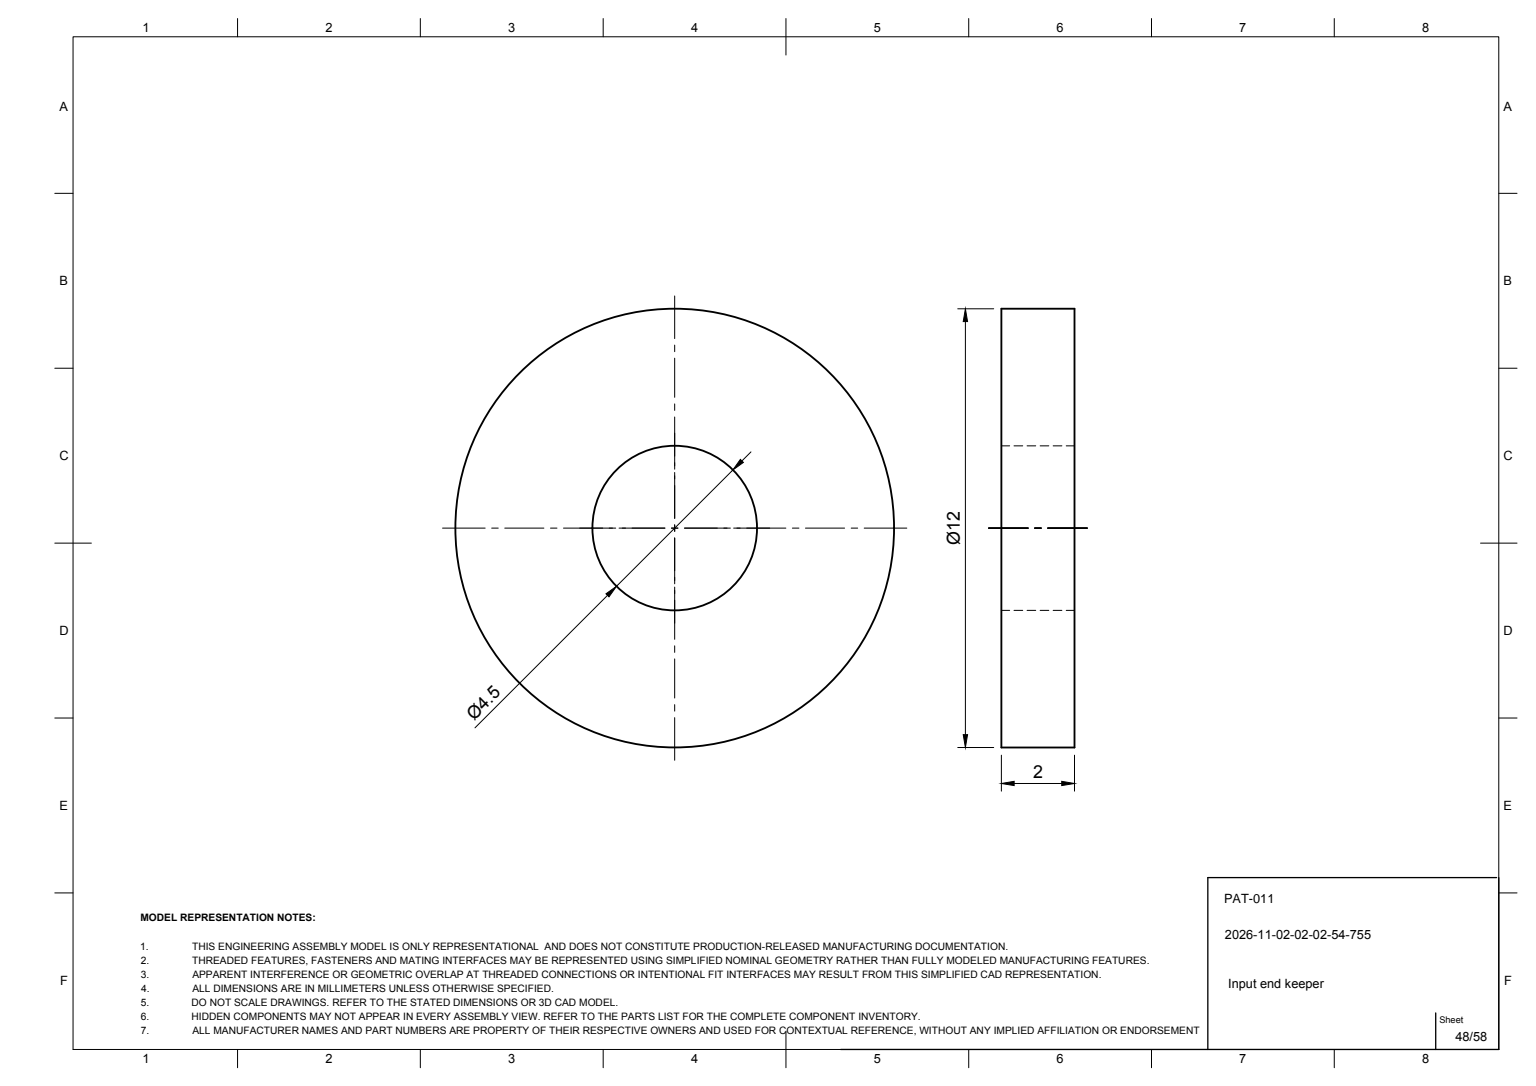
ISO-10303-21;
HEADER;
/* Generated by software containing ST-Developer
 * from STEP Tools, Inc. (www.steptools.com) 
 */

FILE_DESCRIPTION(
/* description */ ('Belt tension measurement rig'),
/* implementation_level */ '2;1');

FILE_NAME(
/* name */ 'Input end keeper.step',
/* time_stamp */ '2026-10-28T03:24:44-07:00',
/* author */ (''),
/* organization */ (''),
/* preprocessor_version */ 'ST-DEVELOPER v20.2',
/* originating_system */ 'Autodesk Translation Framework v15.17.0.0',
/* authorisation */ '');

FILE_SCHEMA (('AUTOMOTIVE_DESIGN { 1 0 10303 214 3 1 1 }'));
ENDSEC;

DATA;
#10=MECHANICAL_DESIGN_GEOMETRIC_PRESENTATION_REPRESENTATION('',(#749),#23587);
#624=SHAPE_REPRESENTATION_RELATIONSHIP('SRR','None',#23874,#679);
#679=ADVANCED_BREP_SHAPE_REPRESENTATION('',(#817),#23572);
#749=STYLED_ITEM('',(#24204),#817);
#817=MANIFOLD_SOLID_BREP('Body1',#12256);
#993=FACE_BOUND('',#2697,.T.);
#994=FACE_BOUND('',#2699,.T.);
#1292=PLANE('',#13869);
#1293=PLANE('',#13870);
#1826=FACE_OUTER_BOUND('',#2694,.T.);
#1827=FACE_OUTER_BOUND('',#2695,.T.);
#1828=FACE_OUTER_BOUND('',#2696,.T.);
#1829=FACE_OUTER_BOUND('',#2698,.T.);
#2694=EDGE_LOOP('',(#9992,#9993,#9994,#9995));
#2695=EDGE_LOOP('',(#9996,#9997,#9998,#9999));
#2696=EDGE_LOOP('',(#10000));
#2697=EDGE_LOOP('',(#10001));
#2698=EDGE_LOOP('',(#10002));
#2699=EDGE_LOOP('',(#10003));
#3505=LINE('',#21539,#4256);
#3506=LINE('',#21545,#4257);
#4256=VECTOR('',#17032,0.225);
#4257=VECTOR('',#17039,0.6);
#4920=CIRCLE('',#13864,0.225);
#4921=CIRCLE('',#13865,0.225);
#4922=CIRCLE('',#13867,0.6);
#4923=CIRCLE('',#13868,0.6);
#5935=VERTEX_POINT('',#21536);
#5936=VERTEX_POINT('',#21538);
#5937=VERTEX_POINT('',#21542);
#5938=VERTEX_POINT('',#21544);
#7355=EDGE_CURVE('',#5935,#5935,#4920,.T.);
#7356=EDGE_CURVE('',#5935,#5936,#3505,.T.);
#7357=EDGE_CURVE('',#5936,#5936,#4921,.T.);
#7358=EDGE_CURVE('',#5937,#5937,#4922,.T.);
#7359=EDGE_CURVE('',#5937,#5938,#3506,.T.);
#7360=EDGE_CURVE('',#5938,#5938,#4923,.T.);
#9992=ORIENTED_EDGE('',*,*,#7355,.F.);
#9993=ORIENTED_EDGE('',*,*,#7356,.T.);
#9994=ORIENTED_EDGE('',*,*,#7357,.T.);
#9995=ORIENTED_EDGE('',*,*,#7356,.F.);
#9996=ORIENTED_EDGE('',*,*,#7358,.F.);
#9997=ORIENTED_EDGE('',*,*,#7359,.T.);
#9998=ORIENTED_EDGE('',*,*,#7360,.T.);
#9999=ORIENTED_EDGE('',*,*,#7359,.F.);
#10000=ORIENTED_EDGE('',*,*,#7358,.T.);
#10001=ORIENTED_EDGE('',*,*,#7355,.T.);
#10002=ORIENTED_EDGE('',*,*,#7360,.F.);
#10003=ORIENTED_EDGE('',*,*,#7357,.F.);
#11329=CYLINDRICAL_SURFACE('',#13863,0.225);
#11330=CYLINDRICAL_SURFACE('',#13866,0.6);
#11967=ADVANCED_FACE('',(#1826),#11329,.F.);
#11968=ADVANCED_FACE('',(#1827),#11330,.T.);
#11969=ADVANCED_FACE('',(#1828,#993),#1292,.T.);
#11970=ADVANCED_FACE('',(#1829,#994),#1293,.F.);
#12256=CLOSED_SHELL('',(#11967,#11968,#11969,#11970));
#13862=AXIS2_PLACEMENT_3D('',#21534,#17026,#17027);
#13863=AXIS2_PLACEMENT_3D('',#21535,#17028,#17029);
#13864=AXIS2_PLACEMENT_3D('',#21537,#17030,#17031);
#13865=AXIS2_PLACEMENT_3D('',#21540,#17033,#17034);
#13866=AXIS2_PLACEMENT_3D('',#21541,#17035,#17036);
#13867=AXIS2_PLACEMENT_3D('',#21543,#17037,#17038);
#13868=AXIS2_PLACEMENT_3D('',#21546,#17040,#17041);
#13869=AXIS2_PLACEMENT_3D('',#21547,#17042,#17043);
#13870=AXIS2_PLACEMENT_3D('',#21548,#17044,#17045);
#17026=DIRECTION('axis',(0.,0.,1.));
#17027=DIRECTION('refdir',(1.,0.,0.));
#17028=DIRECTION('center_axis',(0.,1.,0.));
#17029=DIRECTION('ref_axis',(1.,0.,0.));
#17030=DIRECTION('center_axis',(0.,-1.,0.));
#17031=DIRECTION('ref_axis',(1.,0.,0.));
#17032=DIRECTION('',(0.,-1.,0.));
#17033=DIRECTION('center_axis',(0.,-1.,0.));
#17034=DIRECTION('ref_axis',(1.,0.,0.));
#17035=DIRECTION('center_axis',(0.,1.,0.));
#17036=DIRECTION('ref_axis',(1.,0.,0.));
#17037=DIRECTION('center_axis',(0.,1.,0.));
#17038=DIRECTION('ref_axis',(1.,0.,0.));
#17039=DIRECTION('',(0.,-1.,0.));
#17040=DIRECTION('center_axis',(0.,1.,0.));
#17041=DIRECTION('ref_axis',(1.,0.,0.));
#17042=DIRECTION('center_axis',(0.,1.,0.));
#17043=DIRECTION('ref_axis',(1.,0.,0.));
#17044=DIRECTION('center_axis',(0.,1.,0.));
#17045=DIRECTION('ref_axis',(1.,0.,0.));
#21534=CARTESIAN_POINT('',(0.,0.,0.));
#21535=CARTESIAN_POINT('Origin',(0.,-5.2,7.));
#21536=CARTESIAN_POINT('',(-0.225,-5.,7.));
#21537=CARTESIAN_POINT('Origin',(0.,-5.,7.));
#21538=CARTESIAN_POINT('',(-0.225,-5.2,7.));
#21539=CARTESIAN_POINT('',(-0.225,-5.2,7.));
#21540=CARTESIAN_POINT('Origin',(0.,-5.2,7.));
#21541=CARTESIAN_POINT('Origin',(0.,-5.2,7.));
#21542=CARTESIAN_POINT('',(-0.6,-5.,7.));
#21543=CARTESIAN_POINT('Origin',(0.,-5.,7.));
#21544=CARTESIAN_POINT('',(-0.6,-5.2,7.));
#21545=CARTESIAN_POINT('',(-0.6,-5.2,7.));
#21546=CARTESIAN_POINT('Origin',(0.,-5.2,7.));
#21547=CARTESIAN_POINT('Origin',(0.,-5.,7.));
#21548=CARTESIAN_POINT('Origin',(0.,-5.2,7.));
#23507=UNCERTAINTY_MEASURE_WITH_UNIT(LENGTH_MEASURE(0.001),#23588,
'DISTANCE_ACCURACY_VALUE',
'Maximum model space distance between geometric entities at asserted c
onnectivities');
#23522=UNCERTAINTY_MEASURE_WITH_UNIT(LENGTH_MEASURE(0.001),#23588,
'DISTANCE_ACCURACY_VALUE',
'Maximum model space distance between geometric entities at asserted c
onnectivities');
#23572=(
GEOMETRIC_REPRESENTATION_CONTEXT(3)
GLOBAL_UNCERTAINTY_ASSIGNED_CONTEXT((#23507))
GLOBAL_UNIT_ASSIGNED_CONTEXT((#23588,#23590,#23591))
REPRESENTATION_CONTEXT('','3D')
);
#23587=(
GEOMETRIC_REPRESENTATION_CONTEXT(3)
GLOBAL_UNCERTAINTY_ASSIGNED_CONTEXT((#23522))
GLOBAL_UNIT_ASSIGNED_CONTEXT((#23588,#23590,#23591))
REPRESENTATION_CONTEXT('','3D')
);
#23588=(
LENGTH_UNIT()
NAMED_UNIT(*)
SI_UNIT(.CENTI.,.METRE.)
);
#23590=(
NAMED_UNIT(*)
PLANE_ANGLE_UNIT()
SI_UNIT($,.RADIAN.)
);
#23591=(
NAMED_UNIT(*)
SI_UNIT($,.STERADIAN.)
SOLID_ANGLE_UNIT()
);
#23641=SHAPE_DEFINITION_REPRESENTATION(#23718,#23874);
#23718=PRODUCT_DEFINITION_SHAPE('',$,#23939);
#23874=SHAPE_REPRESENTATION('',(#13862),#23572);
#23889=PRODUCT_DEFINITION_CONTEXT('part definition',#24083,'design');
#23939=PRODUCT_DEFINITION('Input end keeper','Input end keeper',#24003,
#23889);
#24003=PRODUCT_DEFINITION_FORMATION('',$,#24134);
#24083=APPLICATION_CONTEXT(
'Core Data for Automotive Mechanical Design Process');
#24084=PRODUCT_CONTEXT('part definition',#24083,'mechanical');
#24134=PRODUCT('Input end keeper','Input end keeper','Input end keeper',
(#24084));
#24198=COLOUR_RGB('Sky Blue',0.24,0.69,0.87);
#24199=FILL_AREA_STYLE_COLOUR('',#24198);
#24200=FILL_AREA_STYLE('',(#24199));
#24201=SURFACE_STYLE_FILL_AREA(#24200);
#24202=SURFACE_SIDE_STYLE('',(#24201));
#24203=SURFACE_STYLE_USAGE(.BOTH.,#24202);
#24204=PRESENTATION_STYLE_ASSIGNMENT((#24203));
ENDSEC;
END-ISO-10303-21;
